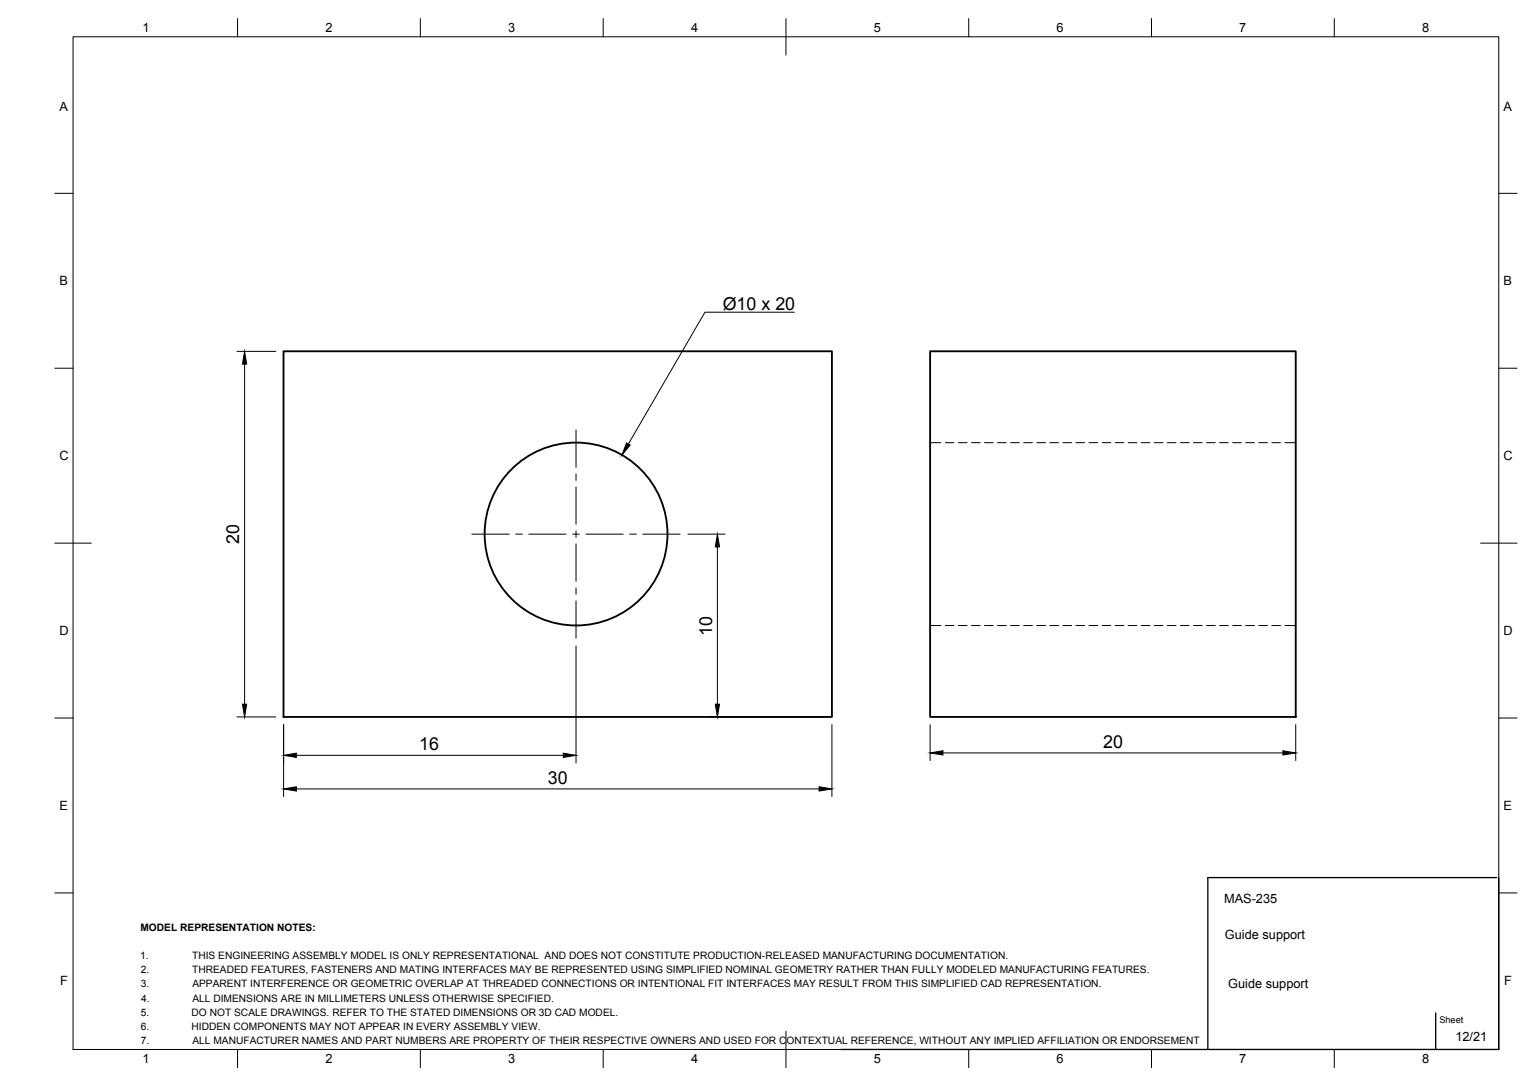
ISO-10303-21;
HEADER;
/* Generated by software containing ST-Developer
 * from STEP Tools, Inc. (www.steptools.com) 
 */

FILE_DESCRIPTION(
/* description */ ('Independent Whitworth quick-return mechanism. Crank radius40, ground-
center spacing80, lever180, connecting rod160, output guide X200. Nomi
nal stroke180 and long/short phase ratio2. Retained guide rods, replac
eable bearing sleeves and captured sliding shoe. No load or production
 rating assigned.'),
/* implementation_level */ '2;1');

FILE_NAME(
/* name */ 'Guide support.step',
/* time_stamp */ '2026-11-09T18:22:56-08:00',
/* author */ (''),
/* organization */ (''),
/* preprocessor_version */ 'ST-DEVELOPER v20.2',
/* originating_system */ 'Autodesk Translation Framework v15.17.0.0',
/* authorisation */ '');

FILE_SCHEMA (('AUTOMOTIVE_DESIGN { 1 0 10303 214 3 1 1 }'));
ENDSEC;

DATA;
#10=MECHANICAL_DESIGN_GEOMETRIC_PRESENTATION_REPRESENTATION('',(#228),#4388);
#188=SHAPE_REPRESENTATION_RELATIONSHIP('SRR','None',#4487,#208);
#208=ADVANCED_BREP_SHAPE_REPRESENTATION('',(#248),#4377);
#228=STYLED_ITEM('',(#4588),#248);
#248=MANIFOLD_SOLID_BREP('Body1',#2333);
#291=FACE_BOUND('',#650,.T.);
#292=FACE_BOUND('',#653,.T.);
#357=PLANE('',#2695);
#358=PLANE('',#2696);
#359=PLANE('',#2697);
#360=PLANE('',#2698);
#361=PLANE('',#2699);
#362=PLANE('',#2700);
#469=FACE_OUTER_BOUND('',#648,.T.);
#470=FACE_OUTER_BOUND('',#649,.T.);
#471=FACE_OUTER_BOUND('',#651,.T.);
#472=FACE_OUTER_BOUND('',#652,.T.);
#473=FACE_OUTER_BOUND('',#654,.T.);
#474=FACE_OUTER_BOUND('',#655,.T.);
#475=FACE_OUTER_BOUND('',#656,.T.);
#648=EDGE_LOOP('',(#1870,#1871,#1872,#1873));
#649=EDGE_LOOP('',(#1874,#1875,#1876,#1877));
#650=EDGE_LOOP('',(#1878));
#651=EDGE_LOOP('',(#1879,#1880,#1881,#1882));
#652=EDGE_LOOP('',(#1883,#1884,#1885,#1886));
#653=EDGE_LOOP('',(#1887));
#654=EDGE_LOOP('',(#1888,#1889,#1890,#1891));
#655=EDGE_LOOP('',(#1892,#1893,#1894,#1895));
#656=EDGE_LOOP('',(#1896,#1897,#1898,#1899));
#845=LINE('',#4009,#984);
#846=LINE('',#4014,#985);
#847=LINE('',#4016,#986);
#848=LINE('',#4018,#987);
#849=LINE('',#4019,#988);
#850=LINE('',#4022,#989);
#851=LINE('',#4024,#990);
#852=LINE('',#4025,#991);
#853=LINE('',#4028,#992);
#854=LINE('',#4030,#993);
#855=LINE('',#4031,#994);
#856=LINE('',#4033,#995);
#857=LINE('',#4034,#996);
#984=VECTOR('',#3241,5.);
#985=VECTOR('',#3246,10.);
#986=VECTOR('',#3247,10.);
#987=VECTOR('',#3248,10.);
#988=VECTOR('',#3249,10.);
#989=VECTOR('',#3252,10.);
#990=VECTOR('',#3253,10.);
#991=VECTOR('',#3254,10.);
#992=VECTOR('',#3257,10.);
#993=VECTOR('',#3258,10.);
#994=VECTOR('',#3259,10.);
#995=VECTOR('',#3262,10.);
#996=VECTOR('',#3263,10.);
#1089=CIRCLE('',#2693,5.);
#1090=CIRCLE('',#2694,5.);
#1251=VERTEX_POINT('',#4006);
#1252=VERTEX_POINT('',#4008);
#1253=VERTEX_POINT('',#4012);
#1254=VERTEX_POINT('',#4013);
#1255=VERTEX_POINT('',#4015);
#1256=VERTEX_POINT('',#4017);
#1257=VERTEX_POINT('',#4021);
#1258=VERTEX_POINT('',#4023);
#1259=VERTEX_POINT('',#4027);
#1260=VERTEX_POINT('',#4029);
#1471=EDGE_CURVE('',#1251,#1251,#1089,.T.);
#1472=EDGE_CURVE('',#1251,#1252,#845,.T.);
#1473=EDGE_CURVE('',#1252,#1252,#1090,.T.);
#1474=EDGE_CURVE('',#1253,#1254,#846,.T.);
#1475=EDGE_CURVE('',#1254,#1255,#847,.T.);
#1476=EDGE_CURVE('',#1256,#1255,#848,.T.);
#1477=EDGE_CURVE('',#1253,#1256,#849,.T.);
#1478=EDGE_CURVE('',#1257,#1253,#850,.T.);
#1479=EDGE_CURVE('',#1258,#1256,#851,.T.);
#1480=EDGE_CURVE('',#1257,#1258,#852,.T.);
#1481=EDGE_CURVE('',#1259,#1257,#853,.T.);
#1482=EDGE_CURVE('',#1260,#1258,#854,.T.);
#1483=EDGE_CURVE('',#1259,#1260,#855,.T.);
#1484=EDGE_CURVE('',#1254,#1259,#856,.T.);
#1485=EDGE_CURVE('',#1255,#1260,#857,.T.);
#1870=ORIENTED_EDGE('',*,*,#1471,.F.);
#1871=ORIENTED_EDGE('',*,*,#1472,.T.);
#1872=ORIENTED_EDGE('',*,*,#1473,.F.);
#1873=ORIENTED_EDGE('',*,*,#1472,.F.);
#1874=ORIENTED_EDGE('',*,*,#1474,.T.);
#1875=ORIENTED_EDGE('',*,*,#1475,.T.);
#1876=ORIENTED_EDGE('',*,*,#1476,.F.);
#1877=ORIENTED_EDGE('',*,*,#1477,.F.);
#1878=ORIENTED_EDGE('',*,*,#1471,.T.);
#1879=ORIENTED_EDGE('',*,*,#1478,.T.);
#1880=ORIENTED_EDGE('',*,*,#1477,.T.);
#1881=ORIENTED_EDGE('',*,*,#1479,.F.);
#1882=ORIENTED_EDGE('',*,*,#1480,.F.);
#1883=ORIENTED_EDGE('',*,*,#1481,.T.);
#1884=ORIENTED_EDGE('',*,*,#1480,.T.);
#1885=ORIENTED_EDGE('',*,*,#1482,.F.);
#1886=ORIENTED_EDGE('',*,*,#1483,.F.);
#1887=ORIENTED_EDGE('',*,*,#1473,.T.);
#1888=ORIENTED_EDGE('',*,*,#1484,.T.);
#1889=ORIENTED_EDGE('',*,*,#1483,.T.);
#1890=ORIENTED_EDGE('',*,*,#1485,.F.);
#1891=ORIENTED_EDGE('',*,*,#1475,.F.);
#1892=ORIENTED_EDGE('',*,*,#1485,.T.);
#1893=ORIENTED_EDGE('',*,*,#1482,.T.);
#1894=ORIENTED_EDGE('',*,*,#1479,.T.);
#1895=ORIENTED_EDGE('',*,*,#1476,.T.);
#1896=ORIENTED_EDGE('',*,*,#1484,.F.);
#1897=ORIENTED_EDGE('',*,*,#1474,.F.);
#1898=ORIENTED_EDGE('',*,*,#1478,.F.);
#1899=ORIENTED_EDGE('',*,*,#1481,.F.);
#2142=CYLINDRICAL_SURFACE('',#2692,5.);
#2241=ADVANCED_FACE('',(#469),#2142,.F.);
#2242=ADVANCED_FACE('',(#470,#291),#357,.T.);
#2243=ADVANCED_FACE('',(#471),#358,.T.);
#2244=ADVANCED_FACE('',(#472,#292),#359,.T.);
#2245=ADVANCED_FACE('',(#473),#360,.T.);
#2246=ADVANCED_FACE('',(#474),#361,.T.);
#2247=ADVANCED_FACE('',(#475),#362,.F.);
#2333=CLOSED_SHELL('',(#2241,#2242,#2243,#2244,#2245,#2246,#2247));
#2691=AXIS2_PLACEMENT_3D('',#4004,#3235,#3236);
#2692=AXIS2_PLACEMENT_3D('',#4005,#3237,#3238);
#2693=AXIS2_PLACEMENT_3D('',#4007,#3239,#3240);
#2694=AXIS2_PLACEMENT_3D('',#4010,#3242,#3243);
#2695=AXIS2_PLACEMENT_3D('',#4011,#3244,#3245);
#2696=AXIS2_PLACEMENT_3D('',#4020,#3250,#3251);
#2697=AXIS2_PLACEMENT_3D('',#4026,#3255,#3256);
#2698=AXIS2_PLACEMENT_3D('',#4032,#3260,#3261);
#2699=AXIS2_PLACEMENT_3D('',#4035,#3264,#3265);
#2700=AXIS2_PLACEMENT_3D('',#4036,#3266,#3267);
#3235=DIRECTION('axis',(0.,0.,1.));
#3236=DIRECTION('refdir',(1.,0.,0.));
#3237=DIRECTION('center_axis',(0.,-1.,0.));
#3238=DIRECTION('ref_axis',(0.,0.,1.));
#3239=DIRECTION('center_axis',(0.,-1.,0.));
#3240=DIRECTION('ref_axis',(0.,0.,1.));
#3241=DIRECTION('',(0.,-1.,0.));
#3242=DIRECTION('center_axis',(0.,1.,0.));
#3243=DIRECTION('ref_axis',(0.,0.,1.));
#3244=DIRECTION('center_axis',(0.,1.,0.));
#3245=DIRECTION('ref_axis',(-1.,0.,0.));
#3246=DIRECTION('',(-1.,0.,0.));
#3247=DIRECTION('',(0.,0.,1.));
#3248=DIRECTION('',(-1.,0.,0.));
#3249=DIRECTION('',(0.,0.,1.));
#3250=DIRECTION('center_axis',(1.,0.,0.));
#3251=DIRECTION('ref_axis',(0.,1.,0.));
#3252=DIRECTION('',(0.,1.,0.));
#3253=DIRECTION('',(0.,1.,0.));
#3254=DIRECTION('',(0.,0.,1.));
#3255=DIRECTION('center_axis',(0.,-1.,0.));
#3256=DIRECTION('ref_axis',(1.,0.,0.));
#3257=DIRECTION('',(1.,0.,0.));
#3258=DIRECTION('',(1.,0.,0.));
#3259=DIRECTION('',(0.,0.,1.));
#3260=DIRECTION('center_axis',(-1.,0.,0.));
#3261=DIRECTION('ref_axis',(0.,-1.,0.));
#3262=DIRECTION('',(0.,-1.,0.));
#3263=DIRECTION('',(0.,-1.,0.));
#3264=DIRECTION('center_axis',(0.,0.,1.));
#3265=DIRECTION('ref_axis',(1.,0.,0.));
#3266=DIRECTION('center_axis',(0.,0.,1.));
#3267=DIRECTION('ref_axis',(1.,0.,0.));
#4004=CARTESIAN_POINT('',(0.,0.,0.));
#4005=CARTESIAN_POINT('Origin',(0.,0.,14.));
#4006=CARTESIAN_POINT('',(6.12323399573677E-16,10.,9.));
#4007=CARTESIAN_POINT('Origin',(0.,10.,14.));
#4008=CARTESIAN_POINT('',(6.12323399573677E-16,-10.,9.));
#4009=CARTESIAN_POINT('',(6.12323399573677E-16,0.,9.));
#4010=CARTESIAN_POINT('Origin',(0.,-10.,14.));
#4011=CARTESIAN_POINT('Origin',(10.,10.,0.));
#4012=CARTESIAN_POINT('',(10.,10.,0.));
#4013=CARTESIAN_POINT('',(-10.,10.,0.));
#4014=CARTESIAN_POINT('',(10.,10.,0.));
#4015=CARTESIAN_POINT('',(-10.,10.,30.));
#4016=CARTESIAN_POINT('',(-10.,10.,0.));
#4017=CARTESIAN_POINT('',(10.,10.,30.));
#4018=CARTESIAN_POINT('',(10.,10.,30.));
#4019=CARTESIAN_POINT('',(10.,10.,0.));
#4020=CARTESIAN_POINT('Origin',(10.,-10.,0.));
#4021=CARTESIAN_POINT('',(10.,-10.,0.));
#4022=CARTESIAN_POINT('',(10.,-10.,0.));
#4023=CARTESIAN_POINT('',(10.,-10.,30.));
#4024=CARTESIAN_POINT('',(10.,-10.,30.));
#4025=CARTESIAN_POINT('',(10.,-10.,0.));
#4026=CARTESIAN_POINT('Origin',(-10.,-10.,0.));
#4027=CARTESIAN_POINT('',(-10.,-10.,0.));
#4028=CARTESIAN_POINT('',(-10.,-10.,0.));
#4029=CARTESIAN_POINT('',(-10.,-10.,30.));
#4030=CARTESIAN_POINT('',(-10.,-10.,30.));
#4031=CARTESIAN_POINT('',(-10.,-10.,0.));
#4032=CARTESIAN_POINT('Origin',(-10.,10.,0.));
#4033=CARTESIAN_POINT('',(-10.,10.,0.));
#4034=CARTESIAN_POINT('',(-10.,10.,30.));
#4035=CARTESIAN_POINT('Origin',(0.,0.,30.));
#4036=CARTESIAN_POINT('Origin',(0.,0.,0.));
#4355=UNCERTAINTY_MEASURE_WITH_UNIT(LENGTH_MEASURE(0.01),#4389,
'DISTANCE_ACCURACY_VALUE',
'Maximum model space distance between geometric entities at asserted c
onnectivities');
#4366=UNCERTAINTY_MEASURE_WITH_UNIT(LENGTH_MEASURE(0.01),#4389,
'DISTANCE_ACCURACY_VALUE',
'Maximum model space distance between geometric entities at asserted c
onnectivities');
#4377=(
GEOMETRIC_REPRESENTATION_CONTEXT(3)
GLOBAL_UNCERTAINTY_ASSIGNED_CONTEXT((#4355))
GLOBAL_UNIT_ASSIGNED_CONTEXT((#4389,#4391,#4392))
REPRESENTATION_CONTEXT('','3D')
);
#4388=(
GEOMETRIC_REPRESENTATION_CONTEXT(3)
GLOBAL_UNCERTAINTY_ASSIGNED_CONTEXT((#4366))
GLOBAL_UNIT_ASSIGNED_CONTEXT((#4389,#4391,#4392))
REPRESENTATION_CONTEXT('','3D')
);
#4389=(
LENGTH_UNIT()
NAMED_UNIT(*)
SI_UNIT(.MILLI.,.METRE.)
);
#4391=(
NAMED_UNIT(*)
PLANE_ANGLE_UNIT()
SI_UNIT($,.RADIAN.)
);
#4392=(
NAMED_UNIT(*)
SI_UNIT($,.STERADIAN.)
SOLID_ANGLE_UNIT()
);
#4403=SHAPE_DEFINITION_REPRESENTATION(#4424,#4487);
#4424=PRODUCT_DEFINITION_SHAPE('',$,#4509);
#4487=SHAPE_REPRESENTATION('',(#2691),#4377);
#4498=PRODUCT_DEFINITION_CONTEXT('part definition',#4563,'design');
#4509=PRODUCT_DEFINITION('Guide support','Guide support',#4530,#4498);
#4530=PRODUCT_DEFINITION_FORMATION('',$,#4575);
#4563=APPLICATION_CONTEXT(
'Core Data for Automotive Mechanical Design Process');
#4564=PRODUCT_CONTEXT('part definition',#4563,'mechanical');
#4575=PRODUCT('Guide support','Guide support',$,(#4564));
#4588=PRESENTATION_STYLE_ASSIGNMENT((#4602));
#4602=SURFACE_STYLE_USAGE(.BOTH.,#4616);
#4616=SURFACE_SIDE_STYLE('',(#4630));
#4630=SURFACE_STYLE_FILL_AREA(#4644);
#4644=FILL_AREA_STYLE('Support gray',(#4658));
#4658=FILL_AREA_STYLE_COLOUR('Support gray',#4672);
#4672=COLOUR_RGB('Support gray',0.407843137254902,0.447058823529412,0.498039215686275);
ENDSEC;
END-ISO-10303-21;
